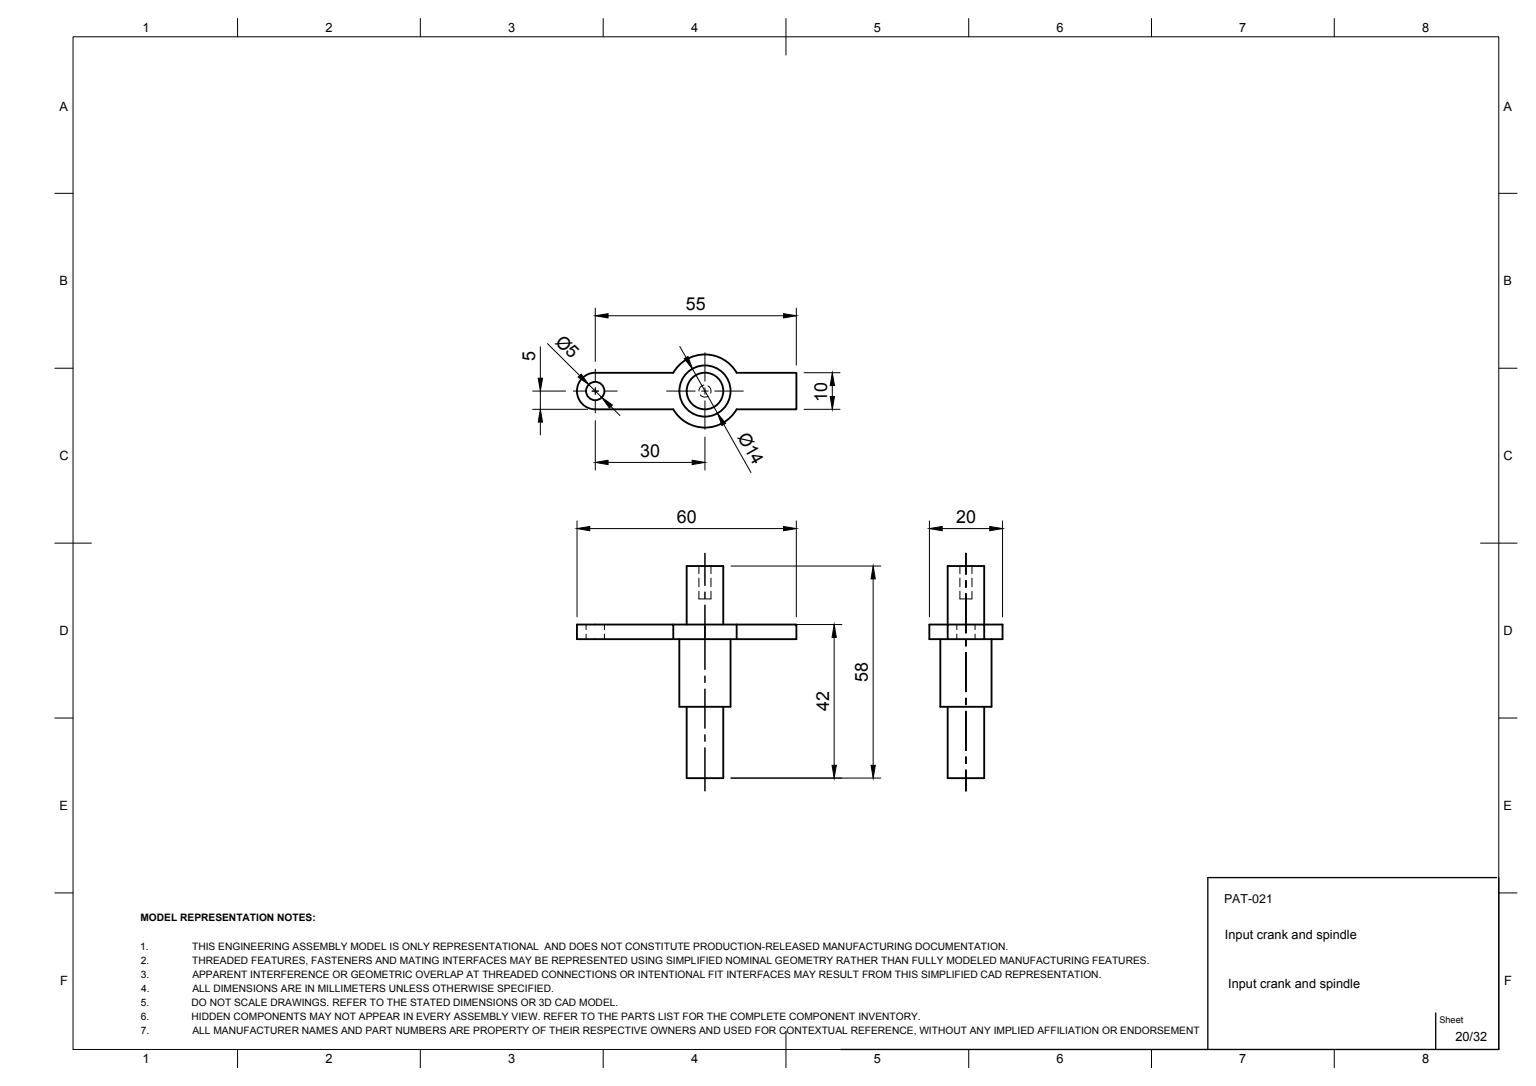
ISO-10303-21;
HEADER;
/* Generated by software containing ST-Developer
 * from STEP Tools, Inc. (www.steptools.com) 
 */

FILE_DESCRIPTION(
/* description */ ('Chain-less indexing wheel (Geneva) drive'),
/* implementation_level */ '2;1');

FILE_NAME(
/* name */ 'Input crank and spindle.step',
/* time_stamp */ '2026-10-28T03:25:22-07:00',
/* author */ (''),
/* organization */ (''),
/* preprocessor_version */ 'ST-DEVELOPER v20.2',
/* originating_system */ 'Autodesk Translation Framework v15.17.0.0',
/* authorisation */ '');

FILE_SCHEMA (('AUTOMOTIVE_DESIGN { 1 0 10303 214 3 1 1 }'));
ENDSEC;

DATA;
#10=MECHANICAL_DESIGN_GEOMETRIC_PRESENTATION_REPRESENTATION('',(#323),#10957);
#265=SHAPE_REPRESENTATION_RELATIONSHIP('SRR','None',#11080,#290);
#290=ADVANCED_BREP_SHAPE_REPRESENTATION('',(#355),#10943);
#323=STYLED_ITEM('',(#11280),#355);
#355=MANIFOLD_SOLID_BREP('Body1',#5720);
#433=FACE_BOUND('',#1232,.T.);
#434=FACE_BOUND('',#1233,.T.);
#435=FACE_BOUND('',#1240,.T.);
#436=FACE_BOUND('',#1241,.T.);
#437=FACE_BOUND('',#1245,.T.);
#438=FACE_BOUND('',#1250,.T.);
#556=PLANE('',#6409);
#557=PLANE('',#6416);
#558=PLANE('',#6420);
#559=PLANE('',#6421);
#560=PLANE('',#6422);
#561=PLANE('',#6423);
#562=PLANE('',#6424);
#563=PLANE('',#6425);
#564=PLANE('',#6431);
#565=PLANE('',#6439);
#566=PLANE('',#6440);
#828=FACE_OUTER_BOUND('',#1227,.T.);
#829=FACE_OUTER_BOUND('',#1228,.T.);
#830=FACE_OUTER_BOUND('',#1229,.T.);
#831=FACE_OUTER_BOUND('',#1230,.T.);
#832=FACE_OUTER_BOUND('',#1231,.T.);
#833=FACE_OUTER_BOUND('',#1234,.T.);
#834=FACE_OUTER_BOUND('',#1235,.T.);
#835=FACE_OUTER_BOUND('',#1236,.T.);
#836=FACE_OUTER_BOUND('',#1237,.T.);
#837=FACE_OUTER_BOUND('',#1238,.T.);
#838=FACE_OUTER_BOUND('',#1239,.T.);
#839=FACE_OUTER_BOUND('',#1242,.T.);
#840=FACE_OUTER_BOUND('',#1243,.T.);
#841=FACE_OUTER_BOUND('',#1244,.T.);
#842=FACE_OUTER_BOUND('',#1246,.T.);
#843=FACE_OUTER_BOUND('',#1247,.T.);
#844=FACE_OUTER_BOUND('',#1248,.T.);
#845=FACE_OUTER_BOUND('',#1249,.T.);
#846=FACE_OUTER_BOUND('',#1251,.T.);
#1227=EDGE_LOOP('',(#4511,#4512,#4513,#4514));
#1228=EDGE_LOOP('',(#4515));
#1229=EDGE_LOOP('',(#4516,#4517,#4518,#4519));
#1230=EDGE_LOOP('',(#4520,#4521,#4522,#4523));
#1231=EDGE_LOOP('',(#4524,#4525,#4526,#4527,#4528,#4529,#4530,#4531));
#1232=EDGE_LOOP('',(#4532));
#1233=EDGE_LOOP('',(#4533));
#1234=EDGE_LOOP('',(#4534,#4535,#4536,#4537));
#1235=EDGE_LOOP('',(#4538,#4539,#4540,#4541));
#1236=EDGE_LOOP('',(#4542,#4543,#4544,#4545));
#1237=EDGE_LOOP('',(#4546,#4547,#4548,#4549));
#1238=EDGE_LOOP('',(#4550,#4551,#4552,#4553));
#1239=EDGE_LOOP('',(#4554,#4555,#4556,#4557,#4558,#4559,#4560,#4561));
#1240=EDGE_LOOP('',(#4562));
#1241=EDGE_LOOP('',(#4563));
#1242=EDGE_LOOP('',(#4564,#4565,#4566,#4567));
#1243=EDGE_LOOP('',(#4568,#4569,#4570,#4571));
#1244=EDGE_LOOP('',(#4572));
#1245=EDGE_LOOP('',(#4573));
#1246=EDGE_LOOP('',(#4574,#4575,#4576,#4577));
#1247=EDGE_LOOP('',(#4578,#4579,#4580,#4581));
#1248=EDGE_LOOP('',(#4582,#4583,#4584,#4585));
#1249=EDGE_LOOP('',(#4586));
#1250=EDGE_LOOP('',(#4587));
#1251=EDGE_LOOP('',(#4588));
#1587=LINE('',#9841,#1961);
#1588=LINE('',#9848,#1962);
#1589=LINE('',#9853,#1963);
#1590=LINE('',#9857,#1964);
#1591=LINE('',#9861,#1965);
#1592=LINE('',#9865,#1966);
#1593=LINE('',#9867,#1967);
#1594=LINE('',#9869,#1968);
#1595=LINE('',#9872,#1969);
#1596=LINE('',#9877,#1970);
#1597=LINE('',#9878,#1971);
#1598=LINE('',#9881,#1972);
#1599=LINE('',#9882,#1973);
#1600=LINE('',#9885,#1974);
#1601=LINE('',#9887,#1975);
#1602=LINE('',#9888,#1976);
#1603=LINE('',#9891,#1977);
#1604=LINE('',#9893,#1978);
#1605=LINE('',#9894,#1979);
#1606=LINE('',#9896,#1980);
#1607=LINE('',#9910,#1981);
#1608=LINE('',#9913,#1982);
#1609=LINE('',#9918,#1983);
#1961=VECTOR('',#7709,0.165);
#1962=VECTOR('',#7718,0.25);
#1963=VECTOR('',#7723,1.);
#1964=VECTOR('',#7726,1.);
#1965=VECTOR('',#7731,1.);
#1966=VECTOR('',#7734,1.);
#1967=VECTOR('',#7735,1.);
#1968=VECTOR('',#7736,1.);
#1969=VECTOR('',#7739,1.);
#1970=VECTOR('',#7744,1.);
#1971=VECTOR('',#7745,1.);
#1972=VECTOR('',#7748,1.);
#1973=VECTOR('',#7749,1.);
#1974=VECTOR('',#7752,1.);
#1975=VECTOR('',#7753,1.);
#1976=VECTOR('',#7754,1.);
#1977=VECTOR('',#7757,1.);
#1978=VECTOR('',#7758,1.);
#1979=VECTOR('',#7759,1.);
#1980=VECTOR('',#7762,1.);
#1981=VECTOR('',#7783,0.7);
#1982=VECTOR('',#7786,0.5);
#1983=VECTOR('',#7793,0.5);
#2369=CIRCLE('',#6407,0.165);
#2370=CIRCLE('',#6408,0.165);
#2371=CIRCLE('',#6411,0.25);
#2372=CIRCLE('',#6412,0.25);
#2373=CIRCLE('',#6414,0.5);
#2374=CIRCLE('',#6415,0.5);
#2375=CIRCLE('',#6417,1.);
#2376=CIRCLE('',#6418,1.);
#2377=CIRCLE('',#6419,0.7);
#2378=CIRCLE('',#6426,1.);
#2379=CIRCLE('',#6427,1.);
#2380=CIRCLE('',#6428,0.5);
#2381=CIRCLE('',#6432,0.7);
#2382=CIRCLE('',#6433,0.5);
#2383=CIRCLE('',#6436,0.5);
#2384=CIRCLE('',#6438,0.5);
#2757=VERTEX_POINT('',#9838);
#2758=VERTEX_POINT('',#9840);
#2759=VERTEX_POINT('',#9845);
#2760=VERTEX_POINT('',#9847);
#2761=VERTEX_POINT('',#9851);
#2762=VERTEX_POINT('',#9852);
#2763=VERTEX_POINT('',#9854);
#2764=VERTEX_POINT('',#9856);
#2765=VERTEX_POINT('',#9860);
#2766=VERTEX_POINT('',#9862);
#2767=VERTEX_POINT('',#9864);
#2768=VERTEX_POINT('',#9866);
#2769=VERTEX_POINT('',#9868);
#2770=VERTEX_POINT('',#9870);
#2771=VERTEX_POINT('',#9873);
#2772=VERTEX_POINT('',#9876);
#2773=VERTEX_POINT('',#9880);
#2774=VERTEX_POINT('',#9884);
#2775=VERTEX_POINT('',#9886);
#2776=VERTEX_POINT('',#9890);
#2777=VERTEX_POINT('',#9892);
#2778=VERTEX_POINT('',#9900);
#2779=VERTEX_POINT('',#9905);
#2780=VERTEX_POINT('',#9907);
#2781=VERTEX_POINT('',#9912);
#2782=VERTEX_POINT('',#9916);
#3381=EDGE_CURVE('',#2757,#2757,#2369,.T.);
#3382=EDGE_CURVE('',#2757,#2758,#1587,.T.);
#3383=EDGE_CURVE('',#2758,#2758,#2370,.T.);
#3384=EDGE_CURVE('',#2759,#2759,#2371,.T.);
#3385=EDGE_CURVE('',#2759,#2760,#1588,.T.);
#3386=EDGE_CURVE('',#2760,#2760,#2372,.T.);
#3387=EDGE_CURVE('',#2761,#2762,#1589,.T.);
#3388=EDGE_CURVE('',#2763,#2762,#2373,.T.);
#3389=EDGE_CURVE('',#2764,#2763,#1590,.T.);
#3390=EDGE_CURVE('',#2764,#2761,#2374,.T.);
#3391=EDGE_CURVE('',#2765,#2764,#1591,.T.);
#3392=EDGE_CURVE('',#2766,#2765,#2375,.T.);
#3393=EDGE_CURVE('',#2767,#2766,#1592,.T.);
#3394=EDGE_CURVE('',#2768,#2767,#1593,.T.);
#3395=EDGE_CURVE('',#2769,#2768,#1594,.T.);
#3396=EDGE_CURVE('',#2770,#2769,#2376,.T.);
#3397=EDGE_CURVE('',#2761,#2770,#1595,.T.);
#3398=EDGE_CURVE('',#2771,#2771,#2377,.T.);
#3399=EDGE_CURVE('',#2772,#2770,#1596,.T.);
#3400=EDGE_CURVE('',#2762,#2772,#1597,.T.);
#3401=EDGE_CURVE('',#2765,#2773,#1598,.T.);
#3402=EDGE_CURVE('',#2773,#2763,#1599,.T.);
#3403=EDGE_CURVE('',#2774,#2766,#1600,.T.);
#3404=EDGE_CURVE('',#2775,#2774,#1601,.T.);
#3405=EDGE_CURVE('',#2767,#2775,#1602,.T.);
#3406=EDGE_CURVE('',#2769,#2776,#1603,.T.);
#3407=EDGE_CURVE('',#2768,#2777,#1604,.T.);
#3408=EDGE_CURVE('',#2776,#2777,#1605,.T.);
#3409=EDGE_CURVE('',#2777,#2775,#1606,.T.);
#3410=EDGE_CURVE('',#2772,#2776,#2378,.T.);
#3411=EDGE_CURVE('',#2774,#2773,#2379,.T.);
#3412=EDGE_CURVE('',#2778,#2778,#2380,.T.);
#3413=EDGE_CURVE('',#2779,#2779,#2381,.T.);
#3414=EDGE_CURVE('',#2780,#2780,#2382,.T.);
#3415=EDGE_CURVE('',#2771,#2779,#1607,.T.);
#3416=EDGE_CURVE('',#2780,#2781,#1608,.T.);
#3417=EDGE_CURVE('',#2781,#2781,#2383,.T.);
#3418=EDGE_CURVE('',#2782,#2782,#2384,.T.);
#3419=EDGE_CURVE('',#2782,#2778,#1609,.T.);
#4511=ORIENTED_EDGE('',*,*,#3381,.F.);
#4512=ORIENTED_EDGE('',*,*,#3382,.T.);
#4513=ORIENTED_EDGE('',*,*,#3383,.F.);
#4514=ORIENTED_EDGE('',*,*,#3382,.F.);
#4515=ORIENTED_EDGE('',*,*,#3381,.T.);
#4516=ORIENTED_EDGE('',*,*,#3384,.F.);
#4517=ORIENTED_EDGE('',*,*,#3385,.T.);
#4518=ORIENTED_EDGE('',*,*,#3386,.F.);
#4519=ORIENTED_EDGE('',*,*,#3385,.F.);
#4520=ORIENTED_EDGE('',*,*,#3387,.T.);
#4521=ORIENTED_EDGE('',*,*,#3388,.F.);
#4522=ORIENTED_EDGE('',*,*,#3389,.F.);
#4523=ORIENTED_EDGE('',*,*,#3390,.T.);
#4524=ORIENTED_EDGE('',*,*,#3391,.F.);
#4525=ORIENTED_EDGE('',*,*,#3392,.F.);
#4526=ORIENTED_EDGE('',*,*,#3393,.F.);
#4527=ORIENTED_EDGE('',*,*,#3394,.F.);
#4528=ORIENTED_EDGE('',*,*,#3395,.F.);
#4529=ORIENTED_EDGE('',*,*,#3396,.F.);
#4530=ORIENTED_EDGE('',*,*,#3397,.F.);
#4531=ORIENTED_EDGE('',*,*,#3390,.F.);
#4532=ORIENTED_EDGE('',*,*,#3384,.T.);
#4533=ORIENTED_EDGE('',*,*,#3398,.T.);
#4534=ORIENTED_EDGE('',*,*,#3399,.F.);
#4535=ORIENTED_EDGE('',*,*,#3400,.F.);
#4536=ORIENTED_EDGE('',*,*,#3387,.F.);
#4537=ORIENTED_EDGE('',*,*,#3397,.T.);
#4538=ORIENTED_EDGE('',*,*,#3401,.F.);
#4539=ORIENTED_EDGE('',*,*,#3391,.T.);
#4540=ORIENTED_EDGE('',*,*,#3389,.T.);
#4541=ORIENTED_EDGE('',*,*,#3402,.F.);
#4542=ORIENTED_EDGE('',*,*,#3403,.F.);
#4543=ORIENTED_EDGE('',*,*,#3404,.F.);
#4544=ORIENTED_EDGE('',*,*,#3405,.F.);
#4545=ORIENTED_EDGE('',*,*,#3393,.T.);
#4546=ORIENTED_EDGE('',*,*,#3406,.F.);
#4547=ORIENTED_EDGE('',*,*,#3395,.T.);
#4548=ORIENTED_EDGE('',*,*,#3407,.T.);
#4549=ORIENTED_EDGE('',*,*,#3408,.F.);
#4550=ORIENTED_EDGE('',*,*,#3394,.T.);
#4551=ORIENTED_EDGE('',*,*,#3405,.T.);
#4552=ORIENTED_EDGE('',*,*,#3409,.F.);
#4553=ORIENTED_EDGE('',*,*,#3407,.F.);
#4554=ORIENTED_EDGE('',*,*,#3400,.T.);
#4555=ORIENTED_EDGE('',*,*,#3410,.T.);
#4556=ORIENTED_EDGE('',*,*,#3408,.T.);
#4557=ORIENTED_EDGE('',*,*,#3409,.T.);
#4558=ORIENTED_EDGE('',*,*,#3404,.T.);
#4559=ORIENTED_EDGE('',*,*,#3411,.T.);
#4560=ORIENTED_EDGE('',*,*,#3402,.T.);
#4561=ORIENTED_EDGE('',*,*,#3388,.T.);
#4562=ORIENTED_EDGE('',*,*,#3386,.T.);
#4563=ORIENTED_EDGE('',*,*,#3412,.F.);
#4564=ORIENTED_EDGE('',*,*,#3403,.T.);
#4565=ORIENTED_EDGE('',*,*,#3392,.T.);
#4566=ORIENTED_EDGE('',*,*,#3401,.T.);
#4567=ORIENTED_EDGE('',*,*,#3411,.F.);
#4568=ORIENTED_EDGE('',*,*,#3406,.T.);
#4569=ORIENTED_EDGE('',*,*,#3410,.F.);
#4570=ORIENTED_EDGE('',*,*,#3399,.T.);
#4571=ORIENTED_EDGE('',*,*,#3396,.T.);
#4572=ORIENTED_EDGE('',*,*,#3413,.F.);
#4573=ORIENTED_EDGE('',*,*,#3414,.F.);
#4574=ORIENTED_EDGE('',*,*,#3398,.F.);
#4575=ORIENTED_EDGE('',*,*,#3415,.T.);
#4576=ORIENTED_EDGE('',*,*,#3413,.T.);
#4577=ORIENTED_EDGE('',*,*,#3415,.F.);
#4578=ORIENTED_EDGE('',*,*,#3414,.T.);
#4579=ORIENTED_EDGE('',*,*,#3416,.T.);
#4580=ORIENTED_EDGE('',*,*,#3417,.T.);
#4581=ORIENTED_EDGE('',*,*,#3416,.F.);
#4582=ORIENTED_EDGE('',*,*,#3418,.F.);
#4583=ORIENTED_EDGE('',*,*,#3419,.T.);
#4584=ORIENTED_EDGE('',*,*,#3412,.T.);
#4585=ORIENTED_EDGE('',*,*,#3419,.F.);
#4586=ORIENTED_EDGE('',*,*,#3418,.T.);
#4587=ORIENTED_EDGE('',*,*,#3383,.T.);
#4588=ORIENTED_EDGE('',*,*,#3417,.F.);
#5309=CYLINDRICAL_SURFACE('',#6406,0.165);
#5310=CYLINDRICAL_SURFACE('',#6410,0.25);
#5311=CYLINDRICAL_SURFACE('',#6413,0.5);
#5312=CYLINDRICAL_SURFACE('',#6429,1.);
#5313=CYLINDRICAL_SURFACE('',#6430,1.);
#5314=CYLINDRICAL_SURFACE('',#6434,0.7);
#5315=CYLINDRICAL_SURFACE('',#6435,0.5);
#5316=CYLINDRICAL_SURFACE('',#6437,0.5);
#5542=ADVANCED_FACE('',(#828),#5309,.F.);
#5543=ADVANCED_FACE('',(#829),#556,.T.);
#5544=ADVANCED_FACE('',(#830),#5310,.F.);
#5545=ADVANCED_FACE('',(#831),#5311,.T.);
#5546=ADVANCED_FACE('',(#832,#433,#434),#557,.F.);
#5547=ADVANCED_FACE('',(#833),#558,.T.);
#5548=ADVANCED_FACE('',(#834),#559,.T.);
#5549=ADVANCED_FACE('',(#835),#560,.T.);
#5550=ADVANCED_FACE('',(#836),#561,.T.);
#5551=ADVANCED_FACE('',(#837),#562,.T.);
#5552=ADVANCED_FACE('',(#838,#435,#436),#563,.T.);
#5553=ADVANCED_FACE('',(#839),#5312,.T.);
#5554=ADVANCED_FACE('',(#840),#5313,.T.);
#5555=ADVANCED_FACE('',(#841,#437),#564,.F.);
#5556=ADVANCED_FACE('',(#842),#5314,.T.);
#5557=ADVANCED_FACE('',(#843),#5315,.T.);
#5558=ADVANCED_FACE('',(#844),#5316,.T.);
#5559=ADVANCED_FACE('',(#845,#438),#565,.T.);
#5560=ADVANCED_FACE('',(#846),#566,.F.);
#5720=CLOSED_SHELL('',(#5542,#5543,#5544,#5545,#5546,#5547,#5548,#5549,
#5550,#5551,#5552,#5553,#5554,#5555,#5556,#5557,#5558,#5559,#5560));
#6405=AXIS2_PLACEMENT_3D('',#9836,#7703,#7704);
#6406=AXIS2_PLACEMENT_3D('',#9837,#7705,#7706);
#6407=AXIS2_PLACEMENT_3D('',#9839,#7707,#7708);
#6408=AXIS2_PLACEMENT_3D('',#9842,#7710,#7711);
#6409=AXIS2_PLACEMENT_3D('',#9843,#7712,#7713);
#6410=AXIS2_PLACEMENT_3D('',#9844,#7714,#7715);
#6411=AXIS2_PLACEMENT_3D('',#9846,#7716,#7717);
#6412=AXIS2_PLACEMENT_3D('',#9849,#7719,#7720);
#6413=AXIS2_PLACEMENT_3D('',#9850,#7721,#7722);
#6414=AXIS2_PLACEMENT_3D('',#9855,#7724,#7725);
#6415=AXIS2_PLACEMENT_3D('',#9858,#7727,#7728);
#6416=AXIS2_PLACEMENT_3D('',#9859,#7729,#7730);
#6417=AXIS2_PLACEMENT_3D('',#9863,#7732,#7733);
#6418=AXIS2_PLACEMENT_3D('',#9871,#7737,#7738);
#6419=AXIS2_PLACEMENT_3D('',#9874,#7740,#7741);
#6420=AXIS2_PLACEMENT_3D('',#9875,#7742,#7743);
#6421=AXIS2_PLACEMENT_3D('',#9879,#7746,#7747);
#6422=AXIS2_PLACEMENT_3D('',#9883,#7750,#7751);
#6423=AXIS2_PLACEMENT_3D('',#9889,#7755,#7756);
#6424=AXIS2_PLACEMENT_3D('',#9895,#7760,#7761);
#6425=AXIS2_PLACEMENT_3D('',#9897,#7763,#7764);
#6426=AXIS2_PLACEMENT_3D('',#9898,#7765,#7766);
#6427=AXIS2_PLACEMENT_3D('',#9899,#7767,#7768);
#6428=AXIS2_PLACEMENT_3D('',#9901,#7769,#7770);
#6429=AXIS2_PLACEMENT_3D('',#9902,#7771,#7772);
#6430=AXIS2_PLACEMENT_3D('',#9903,#7773,#7774);
#6431=AXIS2_PLACEMENT_3D('',#9904,#7775,#7776);
#6432=AXIS2_PLACEMENT_3D('',#9906,#7777,#7778);
#6433=AXIS2_PLACEMENT_3D('',#9908,#7779,#7780);
#6434=AXIS2_PLACEMENT_3D('',#9909,#7781,#7782);
#6435=AXIS2_PLACEMENT_3D('',#9911,#7784,#7785);
#6436=AXIS2_PLACEMENT_3D('',#9914,#7787,#7788);
#6437=AXIS2_PLACEMENT_3D('',#9915,#7789,#7790);
#6438=AXIS2_PLACEMENT_3D('',#9917,#7791,#7792);
#6439=AXIS2_PLACEMENT_3D('',#9919,#7794,#7795);
#6440=AXIS2_PLACEMENT_3D('',#9920,#7796,#7797);
#7703=DIRECTION('axis',(0.,0.,1.));
#7704=DIRECTION('refdir',(1.,0.,0.));
#7705=DIRECTION('center_axis',(0.,0.,1.));
#7706=DIRECTION('ref_axis',(1.,0.,0.));
#7707=DIRECTION('center_axis',(0.,0.,1.));
#7708=DIRECTION('ref_axis',(1.,0.,0.));
#7709=DIRECTION('',(0.,0.,1.));
#7710=DIRECTION('center_axis',(0.,0.,-1.));
#7711=DIRECTION('ref_axis',(1.,0.,0.));
#7712=DIRECTION('center_axis',(0.,0.,1.));
#7713=DIRECTION('ref_axis',(1.,0.,0.));
#7714=DIRECTION('center_axis',(0.,0.,1.));
#7715=DIRECTION('ref_axis',(1.,0.,0.));
#7716=DIRECTION('center_axis',(0.,0.,1.));
#7717=DIRECTION('ref_axis',(1.,0.,0.));
#7718=DIRECTION('',(0.,0.,1.));
#7719=DIRECTION('center_axis',(0.,0.,-1.));
#7720=DIRECTION('ref_axis',(1.,0.,0.));
#7721=DIRECTION('center_axis',(0.,0.,1.));
#7722=DIRECTION('ref_axis',(1.,0.,0.));
#7723=DIRECTION('',(0.,0.,1.));
#7724=DIRECTION('center_axis',(0.,0.,1.));
#7725=DIRECTION('ref_axis',(1.,0.,0.));
#7726=DIRECTION('',(0.,0.,1.));
#7727=DIRECTION('center_axis',(0.,0.,1.));
#7728=DIRECTION('ref_axis',(1.,0.,0.));
#7729=DIRECTION('center_axis',(0.,0.,1.));
#7730=DIRECTION('ref_axis',(1.,0.,0.));
#7731=DIRECTION('',(1.,0.,0.));
#7732=DIRECTION('center_axis',(0.,0.,1.));
#7733=DIRECTION('ref_axis',(1.,0.,0.));
#7734=DIRECTION('',(1.,0.,0.));
#7735=DIRECTION('',(0.,-1.,0.));
#7736=DIRECTION('',(-1.,0.,0.));
#7737=DIRECTION('center_axis',(0.,0.,1.));
#7738=DIRECTION('ref_axis',(1.,0.,0.));
#7739=DIRECTION('',(-1.,0.,0.));
#7740=DIRECTION('center_axis',(0.,0.,1.));
#7741=DIRECTION('ref_axis',(1.,0.,0.));
#7742=DIRECTION('center_axis',(0.,1.,0.));
#7743=DIRECTION('ref_axis',(-1.,0.,0.));
#7744=DIRECTION('',(0.,0.,-1.));
#7745=DIRECTION('',(-1.,0.,0.));
#7746=DIRECTION('center_axis',(0.,-1.,0.));
#7747=DIRECTION('ref_axis',(1.,0.,0.));
#7748=DIRECTION('',(0.,0.,1.));
#7749=DIRECTION('',(1.,0.,0.));
#7750=DIRECTION('center_axis',(0.,-1.,0.));
#7751=DIRECTION('ref_axis',(1.,0.,0.));
#7752=DIRECTION('',(0.,0.,-1.));
#7753=DIRECTION('',(1.,0.,0.));
#7754=DIRECTION('',(0.,0.,1.));
#7755=DIRECTION('center_axis',(0.,1.,0.));
#7756=DIRECTION('ref_axis',(-1.,0.,0.));
#7757=DIRECTION('',(0.,0.,1.));
#7758=DIRECTION('',(0.,0.,1.));
#7759=DIRECTION('',(-1.,0.,0.));
#7760=DIRECTION('center_axis',(-1.,0.,0.));
#7761=DIRECTION('ref_axis',(0.,-1.,0.));
#7762=DIRECTION('',(0.,-1.,0.));
#7763=DIRECTION('center_axis',(0.,0.,1.));
#7764=DIRECTION('ref_axis',(1.,0.,0.));
#7765=DIRECTION('center_axis',(0.,0.,1.));
#7766=DIRECTION('ref_axis',(1.,0.,0.));
#7767=DIRECTION('center_axis',(0.,0.,1.));
#7768=DIRECTION('ref_axis',(1.,0.,0.));
#7769=DIRECTION('center_axis',(0.,0.,1.));
#7770=DIRECTION('ref_axis',(1.,0.,0.));
#7771=DIRECTION('center_axis',(0.,0.,1.));
#7772=DIRECTION('ref_axis',(1.,0.,0.));
#7773=DIRECTION('center_axis',(0.,0.,1.));
#7774=DIRECTION('ref_axis',(1.,0.,0.));
#7775=DIRECTION('center_axis',(0.,0.,1.));
#7776=DIRECTION('ref_axis',(1.,0.,0.));
#7777=DIRECTION('center_axis',(0.,0.,1.));
#7778=DIRECTION('ref_axis',(1.,0.,0.));
#7779=DIRECTION('center_axis',(0.,0.,-1.));
#7780=DIRECTION('ref_axis',(1.,0.,0.));
#7781=DIRECTION('center_axis',(0.,0.,1.));
#7782=DIRECTION('ref_axis',(1.,0.,0.));
#7783=DIRECTION('',(0.,0.,-1.));
#7784=DIRECTION('center_axis',(0.,0.,1.));
#7785=DIRECTION('ref_axis',(1.,0.,0.));
#7786=DIRECTION('',(0.,0.,-1.));
#7787=DIRECTION('center_axis',(0.,0.,1.));
#7788=DIRECTION('ref_axis',(1.,0.,0.));
#7789=DIRECTION('center_axis',(0.,0.,1.));
#7790=DIRECTION('ref_axis',(1.,0.,0.));
#7791=DIRECTION('center_axis',(0.,0.,1.));
#7792=DIRECTION('ref_axis',(1.,0.,0.));
#7793=DIRECTION('',(0.,0.,-1.));
#7794=DIRECTION('center_axis',(0.,0.,1.));
#7795=DIRECTION('ref_axis',(1.,0.,0.));
#7796=DIRECTION('center_axis',(0.,0.,1.));
#7797=DIRECTION('ref_axis',(1.,0.,0.));
#9836=CARTESIAN_POINT('',(0.,0.,0.));
#9837=CARTESIAN_POINT('Origin',(0.,0.,5.9));
#9838=CARTESIAN_POINT('',(-0.165,-2.02066721859313E-17,5.9));
#9839=CARTESIAN_POINT('Origin',(0.,0.,5.9));
#9840=CARTESIAN_POINT('',(-0.165,2.02066721859313E-17,6.8));
#9841=CARTESIAN_POINT('',(-0.165,-2.02066721859313E-17,5.9));
#9842=CARTESIAN_POINT('Origin',(0.,0.,6.8));
#9843=CARTESIAN_POINT('Origin',(0.,0.,5.9));
#9844=CARTESIAN_POINT('Origin',(3.,0.,4.7));
#9845=CARTESIAN_POINT('',(2.75,-3.06161699786838E-17,4.8));
#9846=CARTESIAN_POINT('Origin',(3.,0.,4.8));
#9847=CARTESIAN_POINT('',(2.75,3.06161699786838E-17,5.2));
#9848=CARTESIAN_POINT('',(2.75,-3.06161699786838E-17,4.7));
#9849=CARTESIAN_POINT('Origin',(3.,0.,5.2));
#9850=CARTESIAN_POINT('Origin',(3.,0.,4.8));
#9851=CARTESIAN_POINT('',(3.,0.5,4.8));
#9852=CARTESIAN_POINT('',(3.,0.5,5.2));
#9853=CARTESIAN_POINT('',(3.,0.5,4.8));
#9854=CARTESIAN_POINT('',(3.,-0.5,5.2));
#9855=CARTESIAN_POINT('Origin',(3.,0.,5.2));
#9856=CARTESIAN_POINT('',(3.,-0.5,4.8));
#9857=CARTESIAN_POINT('',(3.,-0.5,4.8));
#9858=CARTESIAN_POINT('Origin',(3.,0.,4.8));
#9859=CARTESIAN_POINT('Origin',(0.,0.,4.8));
#9860=CARTESIAN_POINT('',(0.866025403784439,-0.5,4.8));
#9861=CARTESIAN_POINT('',(-2.5,-0.5,4.8));
#9862=CARTESIAN_POINT('',(-0.866025403784439,-0.5,4.8));
#9863=CARTESIAN_POINT('Origin',(0.,0.,4.8));
#9864=CARTESIAN_POINT('',(-2.5,-0.5,4.8));
#9865=CARTESIAN_POINT('',(-2.5,-0.5,4.8));
#9866=CARTESIAN_POINT('',(-2.5,0.5,4.8));
#9867=CARTESIAN_POINT('',(-2.5,0.5,4.8));
#9868=CARTESIAN_POINT('',(-0.866025403784439,0.5,4.8));
#9869=CARTESIAN_POINT('',(3.,0.5,4.8));
#9870=CARTESIAN_POINT('',(0.866025403784439,0.5,4.8));
#9871=CARTESIAN_POINT('Origin',(0.,0.,4.8));
#9872=CARTESIAN_POINT('',(3.,0.5,4.8));
#9873=CARTESIAN_POINT('',(-0.7,-8.57252759403147E-17,4.8));
#9874=CARTESIAN_POINT('Origin',(0.,0.,4.8));
#9875=CARTESIAN_POINT('Origin',(3.,0.5,4.8));
#9876=CARTESIAN_POINT('',(0.866025403784439,0.5,5.2));
#9877=CARTESIAN_POINT('',(0.866025403784439,0.5,4.8));
#9878=CARTESIAN_POINT('',(3.,0.5,5.2));
#9879=CARTESIAN_POINT('Origin',(-2.5,-0.5,4.8));
#9880=CARTESIAN_POINT('',(0.866025403784439,-0.5,5.2));
#9881=CARTESIAN_POINT('',(0.866025403784439,-0.5,4.8));
#9882=CARTESIAN_POINT('',(-2.5,-0.5,5.2));
#9883=CARTESIAN_POINT('Origin',(-2.5,-0.5,4.8));
#9884=CARTESIAN_POINT('',(-0.866025403784439,-0.5,5.2));
#9885=CARTESIAN_POINT('',(-0.866025403784439,-0.5,4.8));
#9886=CARTESIAN_POINT('',(-2.5,-0.5,5.2));
#9887=CARTESIAN_POINT('',(-2.5,-0.5,5.2));
#9888=CARTESIAN_POINT('',(-2.5,-0.5,4.8));
#9889=CARTESIAN_POINT('Origin',(3.,0.5,4.8));
#9890=CARTESIAN_POINT('',(-0.866025403784439,0.5,5.2));
#9891=CARTESIAN_POINT('',(-0.866025403784439,0.5,4.8));
#9892=CARTESIAN_POINT('',(-2.5,0.5,5.2));
#9893=CARTESIAN_POINT('',(-2.5,0.5,4.8));
#9894=CARTESIAN_POINT('',(3.,0.5,5.2));
#9895=CARTESIAN_POINT('Origin',(-2.5,0.5,4.8));
#9896=CARTESIAN_POINT('',(-2.5,0.5,5.2));
#9897=CARTESIAN_POINT('Origin',(0.,0.,5.2));
#9898=CARTESIAN_POINT('Origin',(0.,0.,5.2));
#9899=CARTESIAN_POINT('Origin',(0.,0.,5.2));
#9900=CARTESIAN_POINT('',(-0.5,-6.12323399573677E-17,5.2));
#9901=CARTESIAN_POINT('Origin',(0.,0.,5.2));
#9902=CARTESIAN_POINT('Origin',(0.,0.,4.8));
#9903=CARTESIAN_POINT('Origin',(0.,0.,4.8));
#9904=CARTESIAN_POINT('Origin',(0.,0.,2.95));
#9905=CARTESIAN_POINT('',(-0.7,-8.57252759403147E-17,2.95));
#9906=CARTESIAN_POINT('Origin',(0.,0.,2.95));
#9907=CARTESIAN_POINT('',(-0.5,6.12323399573677E-17,2.95));
#9908=CARTESIAN_POINT('Origin',(0.,0.,2.95));
#9909=CARTESIAN_POINT('Origin',(0.,0.,2.95));
#9910=CARTESIAN_POINT('',(-0.7,-8.57252759403147E-17,2.95));
#9911=CARTESIAN_POINT('Origin',(0.,0.,1.));
#9912=CARTESIAN_POINT('',(-0.5,-6.12323399573677E-17,1.));
#9913=CARTESIAN_POINT('',(-0.5,-6.12323399573677E-17,1.));
#9914=CARTESIAN_POINT('Origin',(0.,0.,1.));
#9915=CARTESIAN_POINT('Origin',(0.,0.,1.));
#9916=CARTESIAN_POINT('',(-0.5,-6.12323399573677E-17,6.8));
#9917=CARTESIAN_POINT('Origin',(0.,0.,6.8));
#9918=CARTESIAN_POINT('',(-0.5,-6.12323399573677E-17,1.));
#9919=CARTESIAN_POINT('Origin',(0.,0.,6.8));
#9920=CARTESIAN_POINT('Origin',(0.,0.,1.));
#10912=UNCERTAINTY_MEASURE_WITH_UNIT(LENGTH_MEASURE(0.001),#10958,
'DISTANCE_ACCURACY_VALUE',
'Maximum model space distance between geometric entities at asserted c
onnectivities');
#10926=UNCERTAINTY_MEASURE_WITH_UNIT(LENGTH_MEASURE(0.001),#10958,
'DISTANCE_ACCURACY_VALUE',
'Maximum model space distance between geometric entities at asserted c
onnectivities');
#10943=(
GEOMETRIC_REPRESENTATION_CONTEXT(3)
GLOBAL_UNCERTAINTY_ASSIGNED_CONTEXT((#10912))
GLOBAL_UNIT_ASSIGNED_CONTEXT((#10958,#10960,#10961))
REPRESENTATION_CONTEXT('','3D')
);
#10957=(
GEOMETRIC_REPRESENTATION_CONTEXT(3)
GLOBAL_UNCERTAINTY_ASSIGNED_CONTEXT((#10926))
GLOBAL_UNIT_ASSIGNED_CONTEXT((#10958,#10960,#10961))
REPRESENTATION_CONTEXT('','3D')
);
#10958=(
LENGTH_UNIT()
NAMED_UNIT(*)
SI_UNIT(.CENTI.,.METRE.)
);
#10960=(
NAMED_UNIT(*)
PLANE_ANGLE_UNIT()
SI_UNIT($,.RADIAN.)
);
#10961=(
NAMED_UNIT(*)
SI_UNIT($,.STERADIAN.)
SOLID_ANGLE_UNIT()
);
#10978=SHAPE_DEFINITION_REPRESENTATION(#11013,#11080);
#11013=PRODUCT_DEFINITION_SHAPE('',$,#11111);
#11080=SHAPE_REPRESENTATION('',(#6405),#10943);
#11094=PRODUCT_DEFINITION_CONTEXT('part definition',#11186,'design');
#11111=PRODUCT_DEFINITION('Input crank and spindle',
'Input crank and spindle',#11141,#11094);
#11141=PRODUCT_DEFINITION_FORMATION('',$,#11204);
#11186=APPLICATION_CONTEXT(
'Core Data for Automotive Mechanical Design Process');
#11187=PRODUCT_CONTEXT('part definition',#11186,'mechanical');
#11204=PRODUCT('Input crank and spindle','Input crank and spindle',
'Input crank and spindle',(#11187));
#11274=COLOUR_RGB('Sky Blue',0.24,0.69,0.87);
#11275=FILL_AREA_STYLE_COLOUR('',#11274);
#11276=FILL_AREA_STYLE('',(#11275));
#11277=SURFACE_STYLE_FILL_AREA(#11276);
#11278=SURFACE_SIDE_STYLE('',(#11277));
#11279=SURFACE_STYLE_USAGE(.BOTH.,#11278);
#11280=PRESENTATION_STYLE_ASSIGNMENT((#11279));
ENDSEC;
END-ISO-10303-21;
